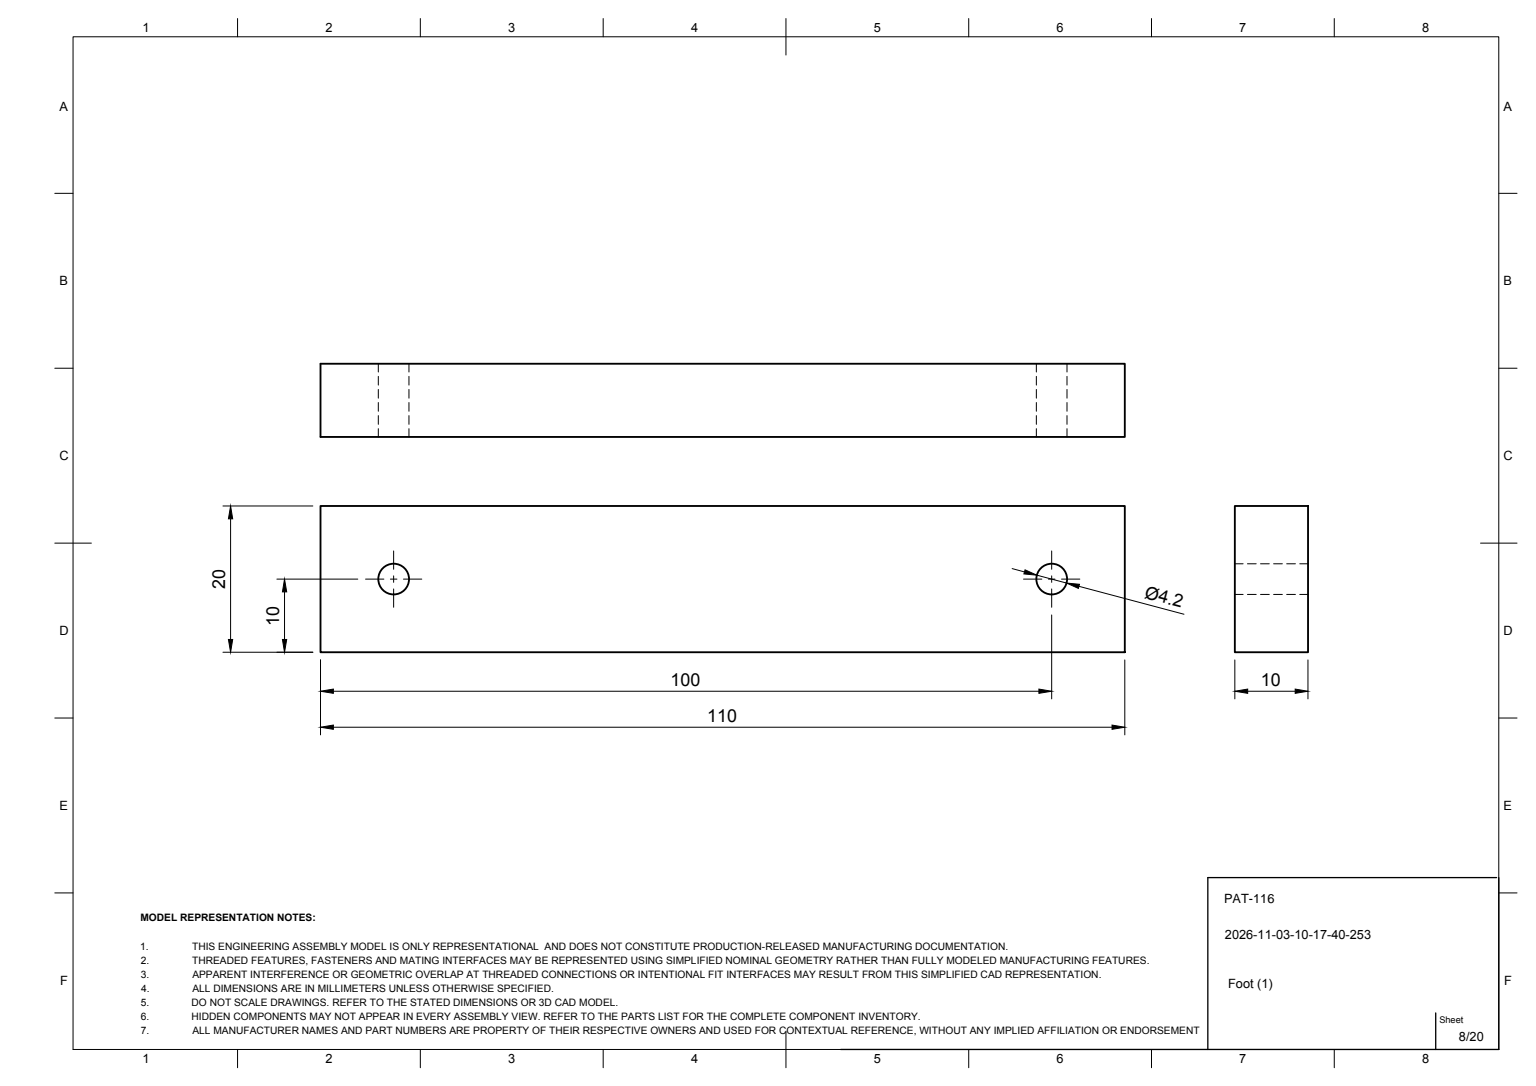
ISO-10303-21;
HEADER;
/* Generated by software containing ST-Developer
 * from STEP Tools, Inc. (www.steptools.com) 
 */

FILE_DESCRIPTION(
/* description */ ('V-block with clamp strap'),
/* implementation_level */ '2;1');

FILE_NAME(
/* name */ 'Foot (1).step',
/* time_stamp */ '2026-10-27T10:50:53-07:00',
/* author */ (''),
/* organization */ (''),
/* preprocessor_version */ 'ST-DEVELOPER v20.2',
/* originating_system */ 'Autodesk Translation Framework v15.17.0.0',
/* authorisation */ '');

FILE_SCHEMA (('AUTOMOTIVE_DESIGN { 1 0 10303 214 3 1 1 }'));
ENDSEC;

DATA;
#10=MECHANICAL_DESIGN_GEOMETRIC_PRESENTATION_REPRESENTATION('',(#269),#7344);
#227=SHAPE_REPRESENTATION_RELATIONSHIP('SRR','None',#7445,#248);
#248=ADVANCED_BREP_SHAPE_REPRESENTATION('',(#290),#7324);
#269=STYLED_ITEM('',(#7645),#290);
#290=MANIFOLD_SOLID_BREP('Body1',#4151);
#335=FACE_BOUND('',#881,.T.);
#336=FACE_BOUND('',#882,.T.);
#337=FACE_BOUND('',#884,.T.);
#338=FACE_BOUND('',#885,.T.);
#404=CIRCLE('',#4481,0.210000000000001);
#405=CIRCLE('',#4482,0.210000000000001);
#406=CIRCLE('',#4484,0.210000000000001);
#407=CIRCLE('',#4485,0.210000000000001);
#519=CYLINDRICAL_SURFACE('',#4480,0.210000000000001);
#520=CYLINDRICAL_SURFACE('',#4483,0.210000000000001);
#604=FACE_OUTER_BOUND('',#874,.T.);
#605=FACE_OUTER_BOUND('',#875,.T.);
#606=FACE_OUTER_BOUND('',#876,.T.);
#607=FACE_OUTER_BOUND('',#877,.T.);
#608=FACE_OUTER_BOUND('',#878,.T.);
#609=FACE_OUTER_BOUND('',#879,.T.);
#610=FACE_OUTER_BOUND('',#880,.T.);
#611=FACE_OUTER_BOUND('',#883,.T.);
#874=EDGE_LOOP('',(#2900,#2901,#2902,#2903));
#875=EDGE_LOOP('',(#2904,#2905,#2906,#2907));
#876=EDGE_LOOP('',(#2908,#2909,#2910,#2911));
#877=EDGE_LOOP('',(#2912,#2913,#2914,#2915));
#878=EDGE_LOOP('',(#2916,#2917,#2918,#2919));
#879=EDGE_LOOP('',(#2920,#2921,#2922,#2923));
#880=EDGE_LOOP('',(#2924,#2925,#2926,#2927));
#881=EDGE_LOOP('',(#2928));
#882=EDGE_LOOP('',(#2929));
#883=EDGE_LOOP('',(#2930,#2931,#2932,#2933));
#884=EDGE_LOOP('',(#2934));
#885=EDGE_LOOP('',(#2935));
#1187=LINE('',#6308,#1552);
#1188=LINE('',#6314,#1553);
#1189=LINE('',#6319,#1554);
#1190=LINE('',#6321,#1555);
#1191=LINE('',#6323,#1556);
#1192=LINE('',#6324,#1557);
#1193=LINE('',#6327,#1558);
#1194=LINE('',#6329,#1559);
#1195=LINE('',#6330,#1560);
#1196=LINE('',#6333,#1561);
#1197=LINE('',#6335,#1562);
#1198=LINE('',#6336,#1563);
#1199=LINE('',#6338,#1564);
#1200=LINE('',#6339,#1565);
#1552=VECTOR('',#5073,0.210000000000001);
#1553=VECTOR('',#5080,0.210000000000001);
#1554=VECTOR('',#5085,1.);
#1555=VECTOR('',#5086,1.);
#1556=VECTOR('',#5087,1.);
#1557=VECTOR('',#5088,1.);
#1558=VECTOR('',#5091,1.);
#1559=VECTOR('',#5092,1.);
#1560=VECTOR('',#5093,1.);
#1561=VECTOR('',#5096,1.);
#1562=VECTOR('',#5097,1.);
#1563=VECTOR('',#5098,1.);
#1564=VECTOR('',#5101,1.);
#1565=VECTOR('',#5102,1.);
#1911=VERTEX_POINT('',#6305);
#1912=VERTEX_POINT('',#6307);
#1913=VERTEX_POINT('',#6311);
#1914=VERTEX_POINT('',#6313);
#1915=VERTEX_POINT('',#6317);
#1916=VERTEX_POINT('',#6318);
#1917=VERTEX_POINT('',#6320);
#1918=VERTEX_POINT('',#6322);
#1919=VERTEX_POINT('',#6326);
#1920=VERTEX_POINT('',#6328);
#1921=VERTEX_POINT('',#6332);
#1922=VERTEX_POINT('',#6334);
#2276=EDGE_CURVE('',#1911,#1911,#404,.T.);
#2277=EDGE_CURVE('',#1911,#1912,#1187,.T.);
#2278=EDGE_CURVE('',#1912,#1912,#405,.T.);
#2279=EDGE_CURVE('',#1913,#1913,#406,.T.);
#2280=EDGE_CURVE('',#1913,#1914,#1188,.T.);
#2281=EDGE_CURVE('',#1914,#1914,#407,.T.);
#2282=EDGE_CURVE('',#1915,#1916,#1189,.T.);
#2283=EDGE_CURVE('',#1916,#1917,#1190,.T.);
#2284=EDGE_CURVE('',#1918,#1917,#1191,.T.);
#2285=EDGE_CURVE('',#1915,#1918,#1192,.T.);
#2286=EDGE_CURVE('',#1919,#1915,#1193,.T.);
#2287=EDGE_CURVE('',#1920,#1918,#1194,.T.);
#2288=EDGE_CURVE('',#1919,#1920,#1195,.T.);
#2289=EDGE_CURVE('',#1921,#1919,#1196,.T.);
#2290=EDGE_CURVE('',#1922,#1920,#1197,.T.);
#2291=EDGE_CURVE('',#1921,#1922,#1198,.T.);
#2292=EDGE_CURVE('',#1916,#1921,#1199,.T.);
#2293=EDGE_CURVE('',#1917,#1922,#1200,.T.);
#2900=ORIENTED_EDGE('',*,*,#2276,.F.);
#2901=ORIENTED_EDGE('',*,*,#2277,.T.);
#2902=ORIENTED_EDGE('',*,*,#2278,.F.);
#2903=ORIENTED_EDGE('',*,*,#2277,.F.);
#2904=ORIENTED_EDGE('',*,*,#2279,.F.);
#2905=ORIENTED_EDGE('',*,*,#2280,.T.);
#2906=ORIENTED_EDGE('',*,*,#2281,.F.);
#2907=ORIENTED_EDGE('',*,*,#2280,.F.);
#2908=ORIENTED_EDGE('',*,*,#2282,.T.);
#2909=ORIENTED_EDGE('',*,*,#2283,.T.);
#2910=ORIENTED_EDGE('',*,*,#2284,.F.);
#2911=ORIENTED_EDGE('',*,*,#2285,.F.);
#2912=ORIENTED_EDGE('',*,*,#2286,.T.);
#2913=ORIENTED_EDGE('',*,*,#2285,.T.);
#2914=ORIENTED_EDGE('',*,*,#2287,.F.);
#2915=ORIENTED_EDGE('',*,*,#2288,.F.);
#2916=ORIENTED_EDGE('',*,*,#2289,.T.);
#2917=ORIENTED_EDGE('',*,*,#2288,.T.);
#2918=ORIENTED_EDGE('',*,*,#2290,.F.);
#2919=ORIENTED_EDGE('',*,*,#2291,.F.);
#2920=ORIENTED_EDGE('',*,*,#2292,.T.);
#2921=ORIENTED_EDGE('',*,*,#2291,.T.);
#2922=ORIENTED_EDGE('',*,*,#2293,.F.);
#2923=ORIENTED_EDGE('',*,*,#2283,.F.);
#2924=ORIENTED_EDGE('',*,*,#2293,.T.);
#2925=ORIENTED_EDGE('',*,*,#2290,.T.);
#2926=ORIENTED_EDGE('',*,*,#2287,.T.);
#2927=ORIENTED_EDGE('',*,*,#2284,.T.);
#2928=ORIENTED_EDGE('',*,*,#2278,.T.);
#2929=ORIENTED_EDGE('',*,*,#2281,.T.);
#2930=ORIENTED_EDGE('',*,*,#2292,.F.);
#2931=ORIENTED_EDGE('',*,*,#2282,.F.);
#2932=ORIENTED_EDGE('',*,*,#2286,.F.);
#2933=ORIENTED_EDGE('',*,*,#2289,.F.);
#2934=ORIENTED_EDGE('',*,*,#2276,.T.);
#2935=ORIENTED_EDGE('',*,*,#2279,.T.);
#3768=PLANE('',#4486);
#3769=PLANE('',#4487);
#3770=PLANE('',#4488);
#3771=PLANE('',#4489);
#3772=PLANE('',#4490);
#3773=PLANE('',#4491);
#3950=ADVANCED_FACE('',(#604),#519,.F.);
#3951=ADVANCED_FACE('',(#605),#520,.F.);
#3952=ADVANCED_FACE('',(#606),#3768,.T.);
#3953=ADVANCED_FACE('',(#607),#3769,.T.);
#3954=ADVANCED_FACE('',(#608),#3770,.T.);
#3955=ADVANCED_FACE('',(#609),#3771,.T.);
#3956=ADVANCED_FACE('',(#610,#335,#336),#3772,.T.);
#3957=ADVANCED_FACE('',(#611,#337,#338),#3773,.F.);
#4151=CLOSED_SHELL('',(#3950,#3951,#3952,#3953,#3954,#3955,#3956,#3957));
#4479=AXIS2_PLACEMENT_3D('',#6303,#5067,#5068);
#4480=AXIS2_PLACEMENT_3D('',#6304,#5069,#5070);
#4481=AXIS2_PLACEMENT_3D('',#6306,#5071,#5072);
#4482=AXIS2_PLACEMENT_3D('',#6309,#5074,#5075);
#4483=AXIS2_PLACEMENT_3D('',#6310,#5076,#5077);
#4484=AXIS2_PLACEMENT_3D('',#6312,#5078,#5079);
#4485=AXIS2_PLACEMENT_3D('',#6315,#5081,#5082);
#4486=AXIS2_PLACEMENT_3D('',#6316,#5083,#5084);
#4487=AXIS2_PLACEMENT_3D('',#6325,#5089,#5090);
#4488=AXIS2_PLACEMENT_3D('',#6331,#5094,#5095);
#4489=AXIS2_PLACEMENT_3D('',#6337,#5099,#5100);
#4490=AXIS2_PLACEMENT_3D('',#6340,#5103,#5104);
#4491=AXIS2_PLACEMENT_3D('',#6341,#5105,#5106);
#5067=DIRECTION('axis',(0.,0.,1.));
#5068=DIRECTION('refdir',(1.,0.,0.));
#5069=DIRECTION('center_axis',(0.,0.,1.));
#5070=DIRECTION('ref_axis',(1.,0.,0.));
#5071=DIRECTION('center_axis',(0.,0.,1.));
#5072=DIRECTION('ref_axis',(1.,0.,0.));
#5073=DIRECTION('',(0.,0.,1.));
#5074=DIRECTION('center_axis',(0.,0.,-1.));
#5075=DIRECTION('ref_axis',(1.,0.,0.));
#5076=DIRECTION('center_axis',(0.,0.,1.));
#5077=DIRECTION('ref_axis',(1.,0.,0.));
#5078=DIRECTION('center_axis',(0.,0.,1.));
#5079=DIRECTION('ref_axis',(1.,0.,0.));
#5080=DIRECTION('',(0.,0.,1.));
#5081=DIRECTION('center_axis',(0.,0.,-1.));
#5082=DIRECTION('ref_axis',(1.,0.,0.));
#5083=DIRECTION('center_axis',(0.,1.,0.));
#5084=DIRECTION('ref_axis',(-1.,0.,0.));
#5085=DIRECTION('',(-1.,0.,0.));
#5086=DIRECTION('',(0.,0.,1.));
#5087=DIRECTION('',(-1.,0.,0.));
#5088=DIRECTION('',(0.,0.,1.));
#5089=DIRECTION('center_axis',(1.,0.,0.));
#5090=DIRECTION('ref_axis',(0.,1.,0.));
#5091=DIRECTION('',(0.,1.,0.));
#5092=DIRECTION('',(0.,1.,0.));
#5093=DIRECTION('',(0.,0.,1.));
#5094=DIRECTION('center_axis',(0.,-1.,0.));
#5095=DIRECTION('ref_axis',(1.,0.,0.));
#5096=DIRECTION('',(1.,0.,0.));
#5097=DIRECTION('',(1.,0.,0.));
#5098=DIRECTION('',(0.,0.,1.));
#5099=DIRECTION('center_axis',(-1.,0.,0.));
#5100=DIRECTION('ref_axis',(0.,-1.,0.));
#5101=DIRECTION('',(0.,-1.,0.));
#5102=DIRECTION('',(0.,-1.,0.));
#5103=DIRECTION('center_axis',(0.,0.,1.));
#5104=DIRECTION('ref_axis',(1.,0.,0.));
#5105=DIRECTION('center_axis',(0.,0.,1.));
#5106=DIRECTION('ref_axis',(1.,0.,0.));
#6303=CARTESIAN_POINT('',(0.,0.,0.));
#6304=CARTESIAN_POINT('Origin',(17.,-4.5,-1.1));
#6305=CARTESIAN_POINT('',(16.79,-4.5,-1.));
#6306=CARTESIAN_POINT('Origin',(17.,-4.5,-1.));
#6307=CARTESIAN_POINT('',(16.79,-4.5,0.));
#6308=CARTESIAN_POINT('',(16.79,-4.5,-1.1));
#6309=CARTESIAN_POINT('Origin',(17.,-4.5,0.));
#6310=CARTESIAN_POINT('Origin',(17.,4.5,-1.1));
#6311=CARTESIAN_POINT('',(16.79,4.5,-1.));
#6312=CARTESIAN_POINT('Origin',(17.,4.5,-1.));
#6313=CARTESIAN_POINT('',(16.79,4.5,0.));
#6314=CARTESIAN_POINT('',(16.79,4.5,-1.1));
#6315=CARTESIAN_POINT('Origin',(17.,4.5,0.));
#6316=CARTESIAN_POINT('Origin',(18.,5.5,-1.));
#6317=CARTESIAN_POINT('',(18.,5.5,-1.));
#6318=CARTESIAN_POINT('',(16.,5.5,-1.));
#6319=CARTESIAN_POINT('',(18.,5.5,-1.));
#6320=CARTESIAN_POINT('',(16.,5.5,0.));
#6321=CARTESIAN_POINT('',(16.,5.5,-1.));
#6322=CARTESIAN_POINT('',(18.,5.5,0.));
#6323=CARTESIAN_POINT('',(18.,5.5,0.));
#6324=CARTESIAN_POINT('',(18.,5.5,-1.));
#6325=CARTESIAN_POINT('Origin',(18.,-5.5,-1.));
#6326=CARTESIAN_POINT('',(18.,-5.5,-1.));
#6327=CARTESIAN_POINT('',(18.,-5.5,-1.));
#6328=CARTESIAN_POINT('',(18.,-5.5,0.));
#6329=CARTESIAN_POINT('',(18.,-5.5,0.));
#6330=CARTESIAN_POINT('',(18.,-5.5,-1.));
#6331=CARTESIAN_POINT('Origin',(16.,-5.5,-1.));
#6332=CARTESIAN_POINT('',(16.,-5.5,-1.));
#6333=CARTESIAN_POINT('',(16.,-5.5,-1.));
#6334=CARTESIAN_POINT('',(16.,-5.5,0.));
#6335=CARTESIAN_POINT('',(16.,-5.5,0.));
#6336=CARTESIAN_POINT('',(16.,-5.5,-1.));
#6337=CARTESIAN_POINT('Origin',(16.,5.5,-1.));
#6338=CARTESIAN_POINT('',(16.,5.5,-1.));
#6339=CARTESIAN_POINT('',(16.,5.5,0.));
#6340=CARTESIAN_POINT('Origin',(17.,0.,0.));
#6341=CARTESIAN_POINT('Origin',(17.,0.,-1.));
#7298=UNCERTAINTY_MEASURE_WITH_UNIT(LENGTH_MEASURE(0.001),#7345,
'DISTANCE_ACCURACY_VALUE',
'Maximum model space distance between geometric entities at asserted c
onnectivities');
#7318=UNCERTAINTY_MEASURE_WITH_UNIT(LENGTH_MEASURE(0.001),#7345,
'DISTANCE_ACCURACY_VALUE',
'Maximum model space distance between geometric entities at asserted c
onnectivities');
#7324=(
GEOMETRIC_REPRESENTATION_CONTEXT(3)
GLOBAL_UNCERTAINTY_ASSIGNED_CONTEXT((#7298))
GLOBAL_UNIT_ASSIGNED_CONTEXT((#7345,#7347,#7348))
REPRESENTATION_CONTEXT('','3D')
);
#7344=(
GEOMETRIC_REPRESENTATION_CONTEXT(3)
GLOBAL_UNCERTAINTY_ASSIGNED_CONTEXT((#7318))
GLOBAL_UNIT_ASSIGNED_CONTEXT((#7345,#7347,#7348))
REPRESENTATION_CONTEXT('','3D')
);
#7345=(
LENGTH_UNIT()
NAMED_UNIT(*)
SI_UNIT(.CENTI.,.METRE.)
);
#7347=(
NAMED_UNIT(*)
PLANE_ANGLE_UNIT()
SI_UNIT($,.RADIAN.)
);
#7348=(
NAMED_UNIT(*)
SI_UNIT($,.STERADIAN.)
SOLID_ANGLE_UNIT()
);
#7354=SHAPE_DEFINITION_REPRESENTATION(#7379,#7445);
#7379=PRODUCT_DEFINITION_SHAPE('',$,#7471);
#7445=SHAPE_REPRESENTATION('',(#4479),#7324);
#7465=PRODUCT_DEFINITION_CONTEXT('part definition',#7542,'design');
#7471=PRODUCT_DEFINITION('Foot (1)','Foot (1)',#7496,#7465);
#7496=PRODUCT_DEFINITION_FORMATION('',$,#7549);
#7542=APPLICATION_CONTEXT(
'Core Data for Automotive Mechanical Design Process');
#7543=PRODUCT_CONTEXT('part definition',#7542,'mechanical');
#7549=PRODUCT('Foot (1)','Foot (1)','Foot (1)',(#7543));
#7639=COLOUR_RGB('Off White',0.89,0.88,0.83);
#7640=FILL_AREA_STYLE_COLOUR('',#7639);
#7641=FILL_AREA_STYLE('',(#7640));
#7642=SURFACE_STYLE_FILL_AREA(#7641);
#7643=SURFACE_SIDE_STYLE('',(#7642));
#7644=SURFACE_STYLE_USAGE(.BOTH.,#7643);
#7645=PRESENTATION_STYLE_ASSIGNMENT((#7644));
ENDSEC;
END-ISO-10303-21;
